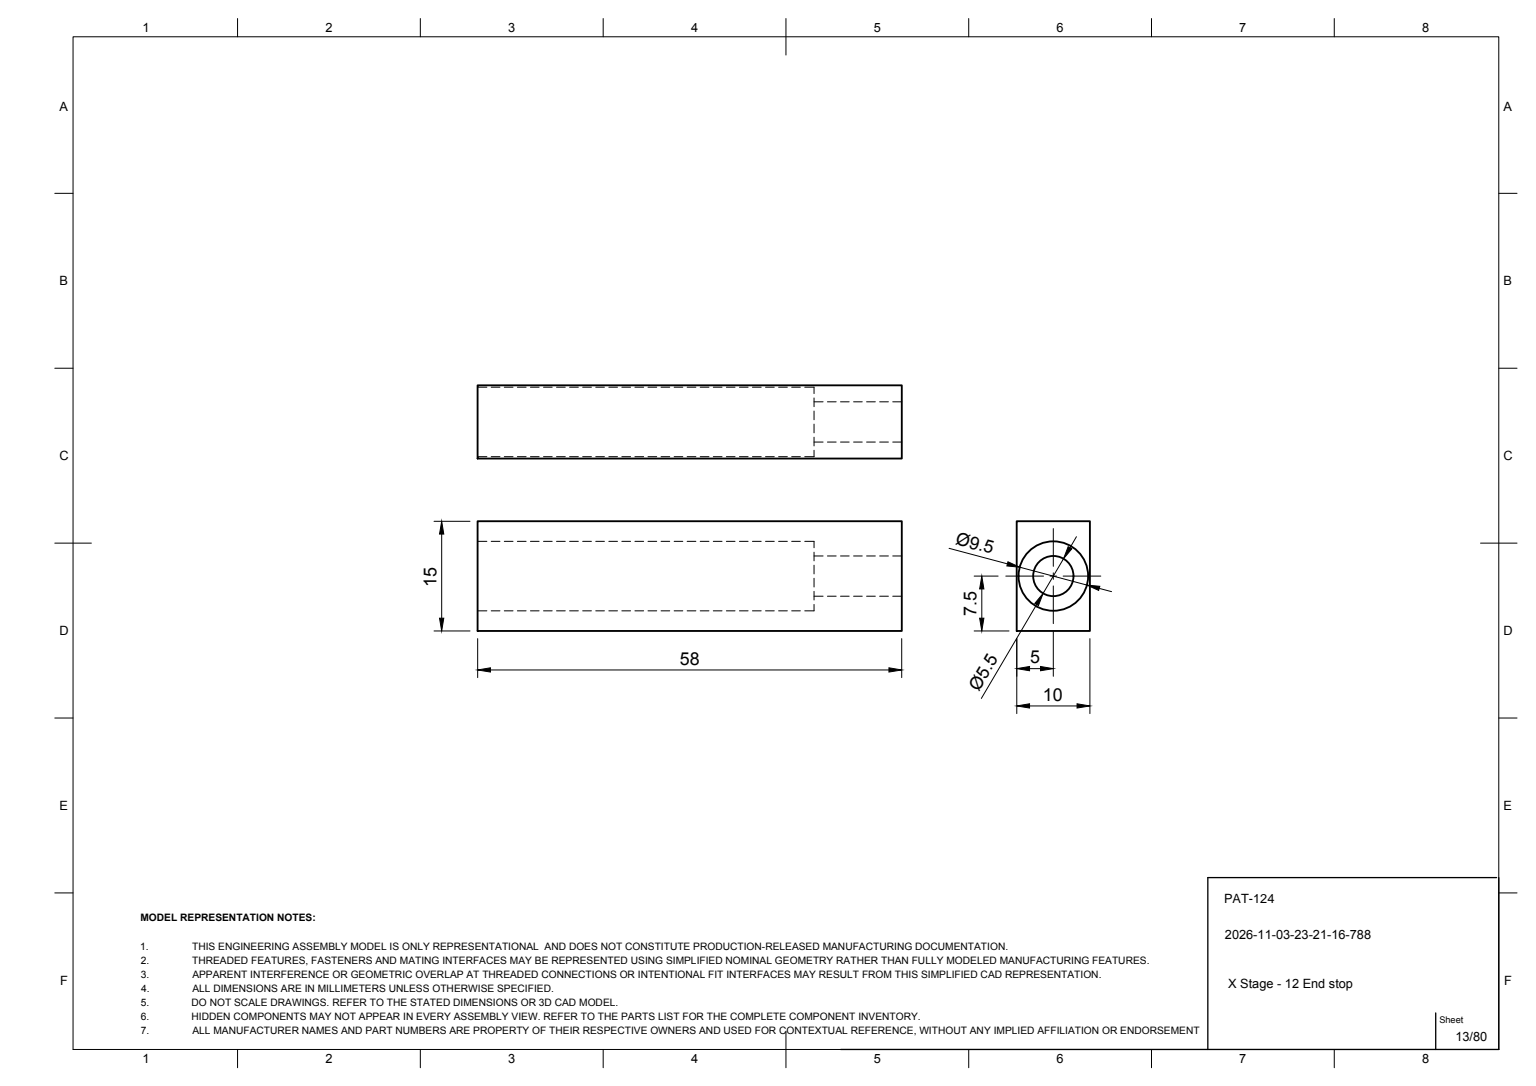
ISO-10303-21;
HEADER;
/* Generated by software containing ST-Developer
 * from STEP Tools, Inc. (www.steptools.com) 
 */

FILE_DESCRIPTION(
/* description */ ('XY cross-slide table'),
/* implementation_level */ '2;1');

FILE_NAME(
/* name */ 'X Stage - 12 End stop.step',
/* time_stamp */ '2026-10-28T03:22:46-07:00',
/* author */ (''),
/* organization */ (''),
/* preprocessor_version */ 'ST-DEVELOPER v20.2',
/* originating_system */ 'Autodesk Translation Framework v15.17.0.0',
/* authorisation */ '');

FILE_SCHEMA (('AUTOMOTIVE_DESIGN { 1 0 10303 214 3 1 1 }'));
ENDSEC;

DATA;
#10=MECHANICAL_DESIGN_GEOMETRIC_PRESENTATION_REPRESENTATION('',(#1678),#62984);
#1512=SHAPE_REPRESENTATION_RELATIONSHIP('SRR','None',#63360,#1595);
#1595=ADVANCED_BREP_SHAPE_REPRESENTATION('',(#1791),#62897);
#1678=STYLED_ITEM('',(#63905),#1791);
#1791=MANIFOLD_SOLID_BREP('Body1',#22972);
#1965=FACE_BOUND('',#4366,.T.);
#1966=FACE_BOUND('',#4373,.T.);
#1967=FACE_BOUND('',#4375,.T.);
#2349=PLANE('',#24218);
#2350=PLANE('',#24222);
#2351=PLANE('',#24223);
#2352=PLANE('',#24224);
#2353=PLANE('',#24225);
#2354=PLANE('',#24226);
#2355=PLANE('',#24227);
#2972=FACE_OUTER_BOUND('',#4364,.T.);
#2973=FACE_OUTER_BOUND('',#4365,.T.);
#2974=FACE_OUTER_BOUND('',#4367,.T.);
#2975=FACE_OUTER_BOUND('',#4368,.T.);
#2976=FACE_OUTER_BOUND('',#4369,.T.);
#2977=FACE_OUTER_BOUND('',#4370,.T.);
#2978=FACE_OUTER_BOUND('',#4371,.T.);
#2979=FACE_OUTER_BOUND('',#4372,.T.);
#2980=FACE_OUTER_BOUND('',#4374,.T.);
#4364=EDGE_LOOP('',(#15362,#15363,#15364,#15365));
#4365=EDGE_LOOP('',(#15366));
#4366=EDGE_LOOP('',(#15367));
#4367=EDGE_LOOP('',(#15368,#15369,#15370,#15371));
#4368=EDGE_LOOP('',(#15372,#15373,#15374,#15375));
#4369=EDGE_LOOP('',(#15376,#15377,#15378,#15379));
#4370=EDGE_LOOP('',(#15380,#15381,#15382,#15383));
#4371=EDGE_LOOP('',(#15384,#15385,#15386,#15387));
#4372=EDGE_LOOP('',(#15388,#15389,#15390,#15391));
#4373=EDGE_LOOP('',(#15392));
#4374=EDGE_LOOP('',(#15393,#15394,#15395,#15396));
#4375=EDGE_LOOP('',(#15397));
#6035=LINE('',#33368,#7522);
#6036=LINE('',#33376,#7523);
#6037=LINE('',#33380,#7524);
#6038=LINE('',#33382,#7525);
#6039=LINE('',#33384,#7526);
#6040=LINE('',#33385,#7527);
#6041=LINE('',#33388,#7528);
#6042=LINE('',#33390,#7529);
#6043=LINE('',#33391,#7530);
#6044=LINE('',#33394,#7531);
#6045=LINE('',#33396,#7532);
#6046=LINE('',#33397,#7533);
#6047=LINE('',#33399,#7534);
#6048=LINE('',#33400,#7535);
#7522=VECTOR('',#27024,0.475);
#7523=VECTOR('',#27035,0.275);
#7524=VECTOR('',#27038,1.);
#7525=VECTOR('',#27039,1.);
#7526=VECTOR('',#27040,1.);
#7527=VECTOR('',#27041,1.);
#7528=VECTOR('',#27044,1.);
#7529=VECTOR('',#27045,1.);
#7530=VECTOR('',#27046,1.);
#7531=VECTOR('',#27049,1.);
#7532=VECTOR('',#27050,1.);
#7533=VECTOR('',#27051,1.);
#7534=VECTOR('',#27054,1.);
#7535=VECTOR('',#27055,1.);
#8980=CIRCLE('',#24216,0.475);
#8981=CIRCLE('',#24217,0.475);
#8982=CIRCLE('',#24219,0.275);
#8983=CIRCLE('',#24221,0.275);
#9923=VERTEX_POINT('',#33365);
#9924=VERTEX_POINT('',#33367);
#9925=VERTEX_POINT('',#33371);
#9926=VERTEX_POINT('',#33374);
#9927=VERTEX_POINT('',#33378);
#9928=VERTEX_POINT('',#33379);
#9929=VERTEX_POINT('',#33381);
#9930=VERTEX_POINT('',#33383);
#9931=VERTEX_POINT('',#33387);
#9932=VERTEX_POINT('',#33389);
#9933=VERTEX_POINT('',#33393);
#9934=VERTEX_POINT('',#33395);
#12065=EDGE_CURVE('',#9923,#9923,#8980,.T.);
#12066=EDGE_CURVE('',#9923,#9924,#6035,.T.);
#12067=EDGE_CURVE('',#9924,#9924,#8981,.T.);
#12068=EDGE_CURVE('',#9925,#9925,#8982,.T.);
#12069=EDGE_CURVE('',#9926,#9926,#8983,.T.);
#12070=EDGE_CURVE('',#9926,#9925,#6036,.T.);
#12071=EDGE_CURVE('',#9927,#9928,#6037,.T.);
#12072=EDGE_CURVE('',#9928,#9929,#6038,.T.);
#12073=EDGE_CURVE('',#9930,#9929,#6039,.T.);
#12074=EDGE_CURVE('',#9927,#9930,#6040,.T.);
#12075=EDGE_CURVE('',#9931,#9927,#6041,.T.);
#12076=EDGE_CURVE('',#9932,#9930,#6042,.T.);
#12077=EDGE_CURVE('',#9931,#9932,#6043,.T.);
#12078=EDGE_CURVE('',#9933,#9931,#6044,.T.);
#12079=EDGE_CURVE('',#9934,#9932,#6045,.T.);
#12080=EDGE_CURVE('',#9933,#9934,#6046,.T.);
#12081=EDGE_CURVE('',#9928,#9933,#6047,.T.);
#12082=EDGE_CURVE('',#9929,#9934,#6048,.T.);
#15362=ORIENTED_EDGE('',*,*,#12065,.F.);
#15363=ORIENTED_EDGE('',*,*,#12066,.T.);
#15364=ORIENTED_EDGE('',*,*,#12067,.F.);
#15365=ORIENTED_EDGE('',*,*,#12066,.F.);
#15366=ORIENTED_EDGE('',*,*,#12065,.T.);
#15367=ORIENTED_EDGE('',*,*,#12068,.F.);
#15368=ORIENTED_EDGE('',*,*,#12069,.F.);
#15369=ORIENTED_EDGE('',*,*,#12070,.T.);
#15370=ORIENTED_EDGE('',*,*,#12068,.T.);
#15371=ORIENTED_EDGE('',*,*,#12070,.F.);
#15372=ORIENTED_EDGE('',*,*,#12071,.T.);
#15373=ORIENTED_EDGE('',*,*,#12072,.T.);
#15374=ORIENTED_EDGE('',*,*,#12073,.F.);
#15375=ORIENTED_EDGE('',*,*,#12074,.F.);
#15376=ORIENTED_EDGE('',*,*,#12075,.T.);
#15377=ORIENTED_EDGE('',*,*,#12074,.T.);
#15378=ORIENTED_EDGE('',*,*,#12076,.F.);
#15379=ORIENTED_EDGE('',*,*,#12077,.F.);
#15380=ORIENTED_EDGE('',*,*,#12078,.T.);
#15381=ORIENTED_EDGE('',*,*,#12077,.T.);
#15382=ORIENTED_EDGE('',*,*,#12079,.F.);
#15383=ORIENTED_EDGE('',*,*,#12080,.F.);
#15384=ORIENTED_EDGE('',*,*,#12081,.T.);
#15385=ORIENTED_EDGE('',*,*,#12080,.T.);
#15386=ORIENTED_EDGE('',*,*,#12082,.F.);
#15387=ORIENTED_EDGE('',*,*,#12072,.F.);
#15388=ORIENTED_EDGE('',*,*,#12082,.T.);
#15389=ORIENTED_EDGE('',*,*,#12079,.T.);
#15390=ORIENTED_EDGE('',*,*,#12076,.T.);
#15391=ORIENTED_EDGE('',*,*,#12073,.T.);
#15392=ORIENTED_EDGE('',*,*,#12067,.T.);
#15393=ORIENTED_EDGE('',*,*,#12081,.F.);
#15394=ORIENTED_EDGE('',*,*,#12071,.F.);
#15395=ORIENTED_EDGE('',*,*,#12075,.F.);
#15396=ORIENTED_EDGE('',*,*,#12078,.F.);
#15397=ORIENTED_EDGE('',*,*,#12069,.T.);
#21090=CYLINDRICAL_SURFACE('',#24215,0.475);
#21091=CYLINDRICAL_SURFACE('',#24220,0.275);
#21753=ADVANCED_FACE('',(#2972),#21090,.F.);
#21754=ADVANCED_FACE('',(#2973,#1965),#2349,.T.);
#21755=ADVANCED_FACE('',(#2974),#21091,.F.);
#21756=ADVANCED_FACE('',(#2975),#2350,.T.);
#21757=ADVANCED_FACE('',(#2976),#2351,.T.);
#21758=ADVANCED_FACE('',(#2977),#2352,.T.);
#21759=ADVANCED_FACE('',(#2978),#2353,.T.);
#21760=ADVANCED_FACE('',(#2979,#1966),#2354,.T.);
#21761=ADVANCED_FACE('',(#2980,#1967),#2355,.F.);
#22972=CLOSED_SHELL('',(#21753,#21754,#21755,#21756,#21757,#21758,#21759,
#21760,#21761));
#24214=AXIS2_PLACEMENT_3D('',#33363,#27018,#27019);
#24215=AXIS2_PLACEMENT_3D('',#33364,#27020,#27021);
#24216=AXIS2_PLACEMENT_3D('',#33366,#27022,#27023);
#24217=AXIS2_PLACEMENT_3D('',#33369,#27025,#27026);
#24218=AXIS2_PLACEMENT_3D('',#33370,#27027,#27028);
#24219=AXIS2_PLACEMENT_3D('',#33372,#27029,#27030);
#24220=AXIS2_PLACEMENT_3D('',#33373,#27031,#27032);
#24221=AXIS2_PLACEMENT_3D('',#33375,#27033,#27034);
#24222=AXIS2_PLACEMENT_3D('',#33377,#27036,#27037);
#24223=AXIS2_PLACEMENT_3D('',#33386,#27042,#27043);
#24224=AXIS2_PLACEMENT_3D('',#33392,#27047,#27048);
#24225=AXIS2_PLACEMENT_3D('',#33398,#27052,#27053);
#24226=AXIS2_PLACEMENT_3D('',#33401,#27056,#27057);
#24227=AXIS2_PLACEMENT_3D('',#33402,#27058,#27059);
#27018=DIRECTION('axis',(0.,0.,1.));
#27019=DIRECTION('refdir',(1.,0.,0.));
#27020=DIRECTION('center_axis',(0.,0.,1.));
#27021=DIRECTION('ref_axis',(1.,0.,0.));
#27022=DIRECTION('center_axis',(0.,0.,1.));
#27023=DIRECTION('ref_axis',(1.,0.,0.));
#27024=DIRECTION('',(0.,0.,1.));
#27025=DIRECTION('center_axis',(0.,0.,-1.));
#27026=DIRECTION('ref_axis',(1.,0.,0.));
#27027=DIRECTION('center_axis',(0.,0.,1.));
#27028=DIRECTION('ref_axis',(1.,0.,0.));
#27029=DIRECTION('center_axis',(0.,0.,1.));
#27030=DIRECTION('ref_axis',(1.,0.,0.));
#27031=DIRECTION('center_axis',(0.,0.,1.));
#27032=DIRECTION('ref_axis',(1.,0.,0.));
#27033=DIRECTION('center_axis',(0.,0.,1.));
#27034=DIRECTION('ref_axis',(1.,0.,0.));
#27035=DIRECTION('',(0.,0.,1.));
#27036=DIRECTION('center_axis',(0.,1.,0.));
#27037=DIRECTION('ref_axis',(-1.,0.,0.));
#27038=DIRECTION('',(-1.,0.,0.));
#27039=DIRECTION('',(0.,0.,1.));
#27040=DIRECTION('',(-1.,0.,0.));
#27041=DIRECTION('',(0.,0.,1.));
#27042=DIRECTION('center_axis',(1.,0.,0.));
#27043=DIRECTION('ref_axis',(0.,1.,0.));
#27044=DIRECTION('',(0.,1.,0.));
#27045=DIRECTION('',(0.,1.,0.));
#27046=DIRECTION('',(0.,0.,1.));
#27047=DIRECTION('center_axis',(0.,-1.,0.));
#27048=DIRECTION('ref_axis',(1.,0.,0.));
#27049=DIRECTION('',(1.,0.,0.));
#27050=DIRECTION('',(1.,0.,0.));
#27051=DIRECTION('',(0.,0.,1.));
#27052=DIRECTION('center_axis',(-1.,0.,0.));
#27053=DIRECTION('ref_axis',(0.,-1.,0.));
#27054=DIRECTION('',(0.,-1.,0.));
#27055=DIRECTION('',(0.,-1.,0.));
#27056=DIRECTION('center_axis',(0.,0.,1.));
#27057=DIRECTION('ref_axis',(1.,0.,0.));
#27058=DIRECTION('center_axis',(0.,0.,1.));
#27059=DIRECTION('ref_axis',(1.,0.,0.));
#33363=CARTESIAN_POINT('',(0.,0.,0.));
#33364=CARTESIAN_POINT('Origin',(3.5,-9.25,2.4));
#33365=CARTESIAN_POINT('',(3.025,-9.25,2.4));
#33366=CARTESIAN_POINT('Origin',(3.5,-9.25,2.4));
#33367=CARTESIAN_POINT('',(3.025,-9.25,7.));
#33368=CARTESIAN_POINT('',(3.025,-9.25,2.4));
#33369=CARTESIAN_POINT('Origin',(3.5,-9.25,7.));
#33370=CARTESIAN_POINT('Origin',(3.5,-9.25,2.4));
#33371=CARTESIAN_POINT('',(3.225,-9.25,2.4));
#33372=CARTESIAN_POINT('Origin',(3.5,-9.25,2.4));
#33373=CARTESIAN_POINT('Origin',(3.5,-9.25,1.1));
#33374=CARTESIAN_POINT('',(3.225,-9.25,1.2));
#33375=CARTESIAN_POINT('Origin',(3.5,-9.25,1.2));
#33376=CARTESIAN_POINT('',(3.225,-9.25,1.1));
#33377=CARTESIAN_POINT('Origin',(4.,-8.5,1.2));
#33378=CARTESIAN_POINT('',(4.,-8.5,1.2));
#33379=CARTESIAN_POINT('',(3.,-8.5,1.2));
#33380=CARTESIAN_POINT('',(4.,-8.5,1.2));
#33381=CARTESIAN_POINT('',(3.,-8.5,7.));
#33382=CARTESIAN_POINT('',(3.,-8.5,1.2));
#33383=CARTESIAN_POINT('',(4.,-8.5,7.));
#33384=CARTESIAN_POINT('',(4.,-8.5,7.));
#33385=CARTESIAN_POINT('',(4.,-8.5,1.2));
#33386=CARTESIAN_POINT('Origin',(4.,-10.,1.2));
#33387=CARTESIAN_POINT('',(4.,-10.,1.2));
#33388=CARTESIAN_POINT('',(4.,-10.,1.2));
#33389=CARTESIAN_POINT('',(4.,-10.,7.));
#33390=CARTESIAN_POINT('',(4.,-10.,7.));
#33391=CARTESIAN_POINT('',(4.,-10.,1.2));
#33392=CARTESIAN_POINT('Origin',(3.,-10.,1.2));
#33393=CARTESIAN_POINT('',(3.,-10.,1.2));
#33394=CARTESIAN_POINT('',(3.,-10.,1.2));
#33395=CARTESIAN_POINT('',(3.,-10.,7.));
#33396=CARTESIAN_POINT('',(3.,-10.,7.));
#33397=CARTESIAN_POINT('',(3.,-10.,1.2));
#33398=CARTESIAN_POINT('Origin',(3.,-8.5,1.2));
#33399=CARTESIAN_POINT('',(3.,-8.5,1.2));
#33400=CARTESIAN_POINT('',(3.,-8.5,7.));
#33401=CARTESIAN_POINT('Origin',(3.5,-9.25,7.));
#33402=CARTESIAN_POINT('Origin',(3.5,-9.25,1.2));
#62798=UNCERTAINTY_MEASURE_WITH_UNIT(LENGTH_MEASURE(0.001),#62985,
'DISTANCE_ACCURACY_VALUE',
'Maximum model space distance between geometric entities at asserted c
onnectivities');
#62885=UNCERTAINTY_MEASURE_WITH_UNIT(LENGTH_MEASURE(0.001),#62985,
'DISTANCE_ACCURACY_VALUE',
'Maximum model space distance between geometric entities at asserted c
onnectivities');
#62897=(
GEOMETRIC_REPRESENTATION_CONTEXT(3)
GLOBAL_UNCERTAINTY_ASSIGNED_CONTEXT((#62798))
GLOBAL_UNIT_ASSIGNED_CONTEXT((#62985,#62987,#62988))
REPRESENTATION_CONTEXT('','3D')
);
#62984=(
GEOMETRIC_REPRESENTATION_CONTEXT(3)
GLOBAL_UNCERTAINTY_ASSIGNED_CONTEXT((#62885))
GLOBAL_UNIT_ASSIGNED_CONTEXT((#62985,#62987,#62988))
REPRESENTATION_CONTEXT('','3D')
);
#62985=(
LENGTH_UNIT()
NAMED_UNIT(*)
SI_UNIT(.CENTI.,.METRE.)
);
#62987=(
NAMED_UNIT(*)
PLANE_ANGLE_UNIT()
SI_UNIT($,.RADIAN.)
);
#62988=(
NAMED_UNIT(*)
SI_UNIT($,.STERADIAN.)
SOLID_ANGLE_UNIT()
);
#63000=SHAPE_DEFINITION_REPRESENTATION(#63098,#63360);
#63098=PRODUCT_DEFINITION_SHAPE('',$,#63459);
#63360=SHAPE_REPRESENTATION('',(#24214),#62897);
#63447=PRODUCT_DEFINITION_CONTEXT('part definition',#63743,'design');
#63459=PRODUCT_DEFINITION('X Stage - 12 End stop',
'X Stage - 12 End stop',#63557,#63447);
#63557=PRODUCT_DEFINITION_FORMATION('',$,#63756);
#63743=APPLICATION_CONTEXT(
'Core Data for Automotive Mechanical Design Process');
#63744=PRODUCT_CONTEXT('part definition',#63743,'mechanical');
#63756=PRODUCT('X Stage - 12 End stop','X Stage - 12 End stop',
'X Stage - 12 End stop',(#63744));
#63899=COLOUR_RGB('Sky Blue',0.24,0.69,0.87);
#63900=FILL_AREA_STYLE_COLOUR('',#63899);
#63901=FILL_AREA_STYLE('',(#63900));
#63902=SURFACE_STYLE_FILL_AREA(#63901);
#63903=SURFACE_SIDE_STYLE('',(#63902));
#63904=SURFACE_STYLE_USAGE(.BOTH.,#63903);
#63905=PRESENTATION_STYLE_ASSIGNMENT((#63904));
ENDSEC;
END-ISO-10303-21;
